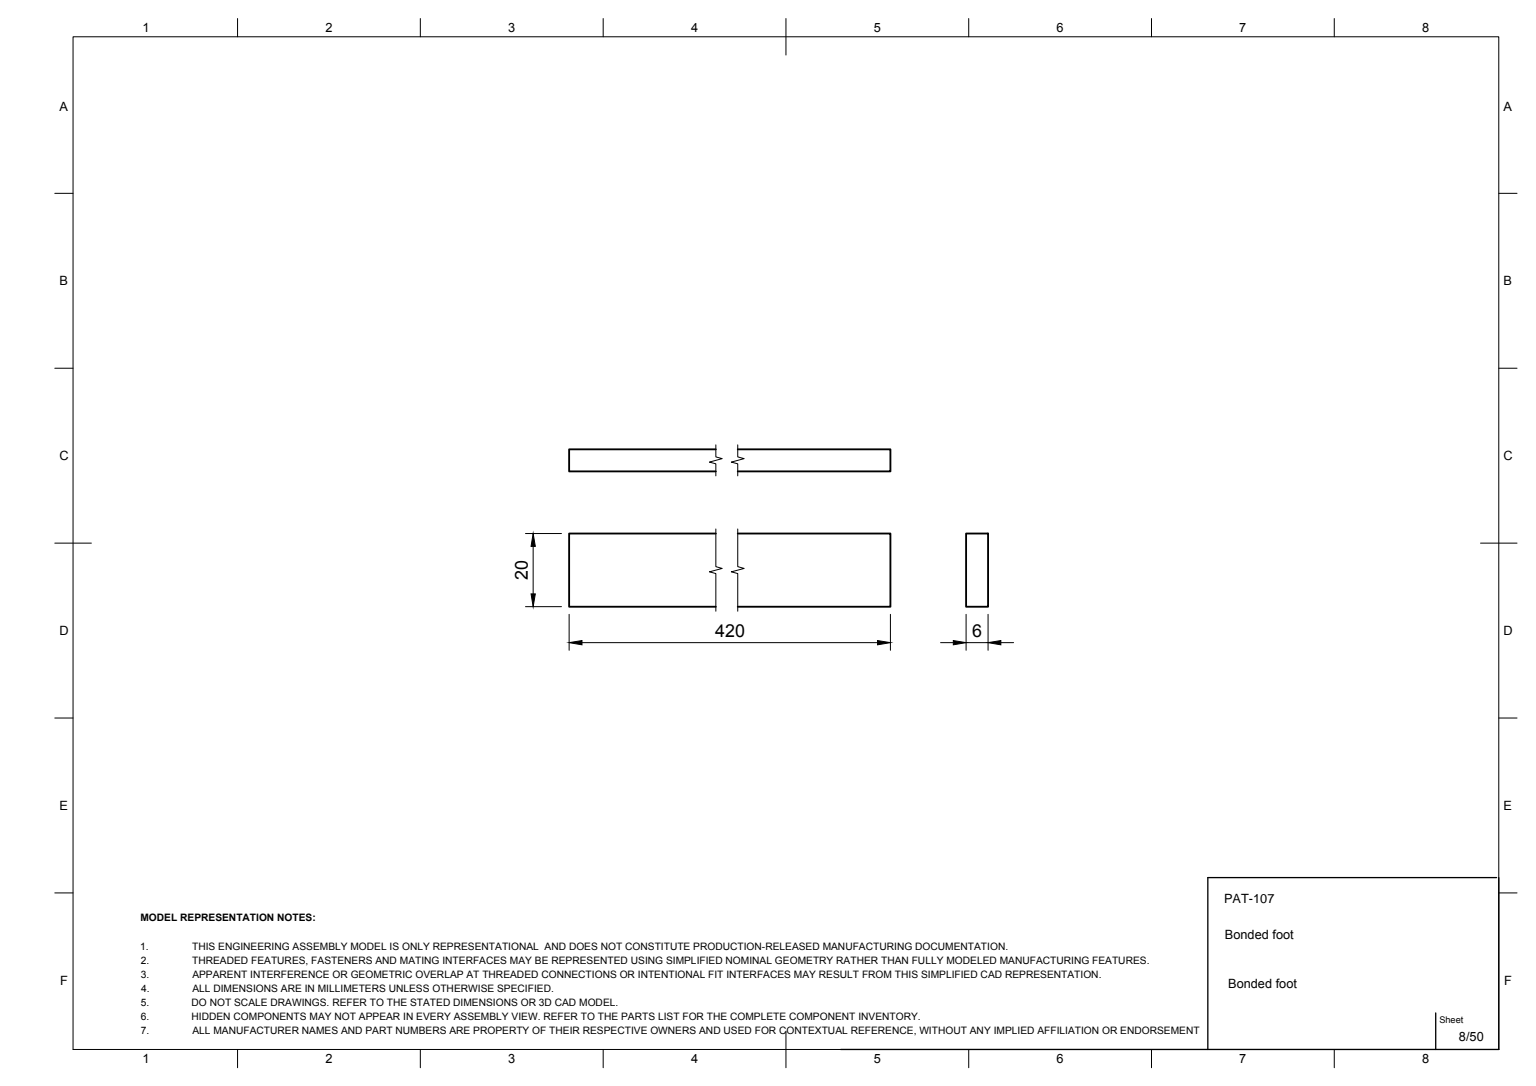
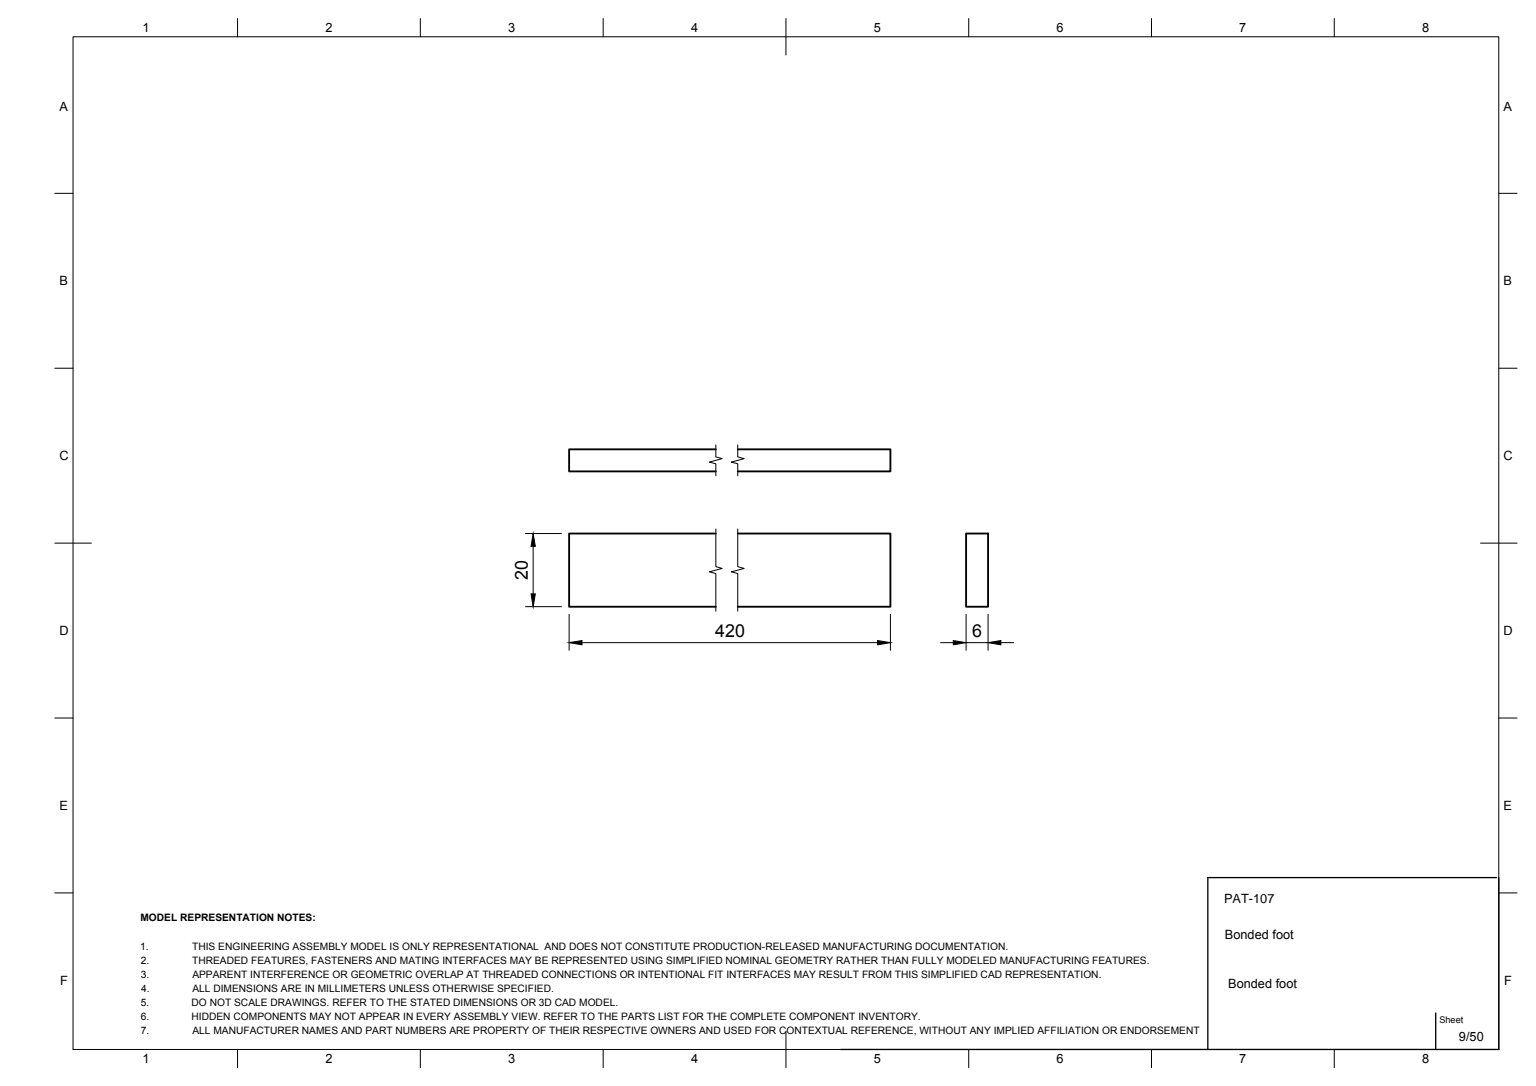
ISO-10303-21;
HEADER;
/* Generated by software containing ST-Developer
 * from STEP Tools, Inc. (www.steptools.com) 
 */

FILE_DESCRIPTION(
/* description */ ('Turntable on roller ring'),
/* implementation_level */ '2;1');

FILE_NAME(
/* name */ 'Bonded foot.step',
/* time_stamp */ '2026-10-28T03:23:59-07:00',
/* author */ (''),
/* organization */ (''),
/* preprocessor_version */ 'ST-DEVELOPER v20.2',
/* originating_system */ 'Autodesk Translation Framework v15.17.0.0',
/* authorisation */ '');

FILE_SCHEMA (('AUTOMOTIVE_DESIGN { 1 0 10303 214 3 1 1 }'));
ENDSEC;

DATA;
#10=MECHANICAL_DESIGN_GEOMETRIC_PRESENTATION_REPRESENTATION('',(#635),#16281);
#516=SHAPE_REPRESENTATION_RELATIONSHIP('SRR','None',#16531,#571);
#571=ADVANCED_BREP_SHAPE_REPRESENTATION('',(#706),#16225);
#635=STYLED_ITEM('',(#16946),#706);
#706=MANIFOLD_SOLID_BREP('Body1',#8377);
#1039=PLANE('',#9375);
#1040=PLANE('',#9376);
#1041=PLANE('',#9377);
#1042=PLANE('',#9378);
#1043=PLANE('',#9379);
#1044=PLANE('',#9380);
#1386=FACE_OUTER_BOUND('',#1967,.T.);
#1387=FACE_OUTER_BOUND('',#1968,.T.);
#1388=FACE_OUTER_BOUND('',#1969,.T.);
#1389=FACE_OUTER_BOUND('',#1970,.T.);
#1390=FACE_OUTER_BOUND('',#1971,.T.);
#1391=FACE_OUTER_BOUND('',#1972,.T.);
#1967=EDGE_LOOP('',(#6245,#6246,#6247,#6248));
#1968=EDGE_LOOP('',(#6249,#6250,#6251,#6252));
#1969=EDGE_LOOP('',(#6253,#6254,#6255,#6256));
#1970=EDGE_LOOP('',(#6257,#6258,#6259,#6260));
#1971=EDGE_LOOP('',(#6261,#6262,#6263,#6264));
#1972=EDGE_LOOP('',(#6265,#6266,#6267,#6268));
#2594=LINE('',#14042,#3077);
#2595=LINE('',#14044,#3078);
#2596=LINE('',#14046,#3079);
#2597=LINE('',#14047,#3080);
#2598=LINE('',#14050,#3081);
#2599=LINE('',#14052,#3082);
#2600=LINE('',#14053,#3083);
#2601=LINE('',#14056,#3084);
#2602=LINE('',#14058,#3085);
#2603=LINE('',#14059,#3086);
#2604=LINE('',#14061,#3087);
#2605=LINE('',#14062,#3088);
#3077=VECTOR('',#10973,1.);
#3078=VECTOR('',#10974,1.);
#3079=VECTOR('',#10975,1.);
#3080=VECTOR('',#10976,1.);
#3081=VECTOR('',#10979,1.);
#3082=VECTOR('',#10980,1.);
#3083=VECTOR('',#10981,1.);
#3084=VECTOR('',#10984,1.);
#3085=VECTOR('',#10985,1.);
#3086=VECTOR('',#10986,1.);
#3087=VECTOR('',#10989,1.);
#3088=VECTOR('',#10990,1.);
#4153=VERTEX_POINT('',#14040);
#4154=VERTEX_POINT('',#14041);
#4155=VERTEX_POINT('',#14043);
#4156=VERTEX_POINT('',#14045);
#4157=VERTEX_POINT('',#14049);
#4158=VERTEX_POINT('',#14051);
#4159=VERTEX_POINT('',#14055);
#4160=VERTEX_POINT('',#14057);
#4933=EDGE_CURVE('',#4153,#4154,#2594,.T.);
#4934=EDGE_CURVE('',#4154,#4155,#2595,.T.);
#4935=EDGE_CURVE('',#4156,#4155,#2596,.T.);
#4936=EDGE_CURVE('',#4153,#4156,#2597,.T.);
#4937=EDGE_CURVE('',#4157,#4153,#2598,.T.);
#4938=EDGE_CURVE('',#4158,#4156,#2599,.T.);
#4939=EDGE_CURVE('',#4157,#4158,#2600,.T.);
#4940=EDGE_CURVE('',#4159,#4157,#2601,.T.);
#4941=EDGE_CURVE('',#4160,#4158,#2602,.T.);
#4942=EDGE_CURVE('',#4159,#4160,#2603,.T.);
#4943=EDGE_CURVE('',#4154,#4159,#2604,.T.);
#4944=EDGE_CURVE('',#4155,#4160,#2605,.T.);
#6245=ORIENTED_EDGE('',*,*,#4933,.T.);
#6246=ORIENTED_EDGE('',*,*,#4934,.T.);
#6247=ORIENTED_EDGE('',*,*,#4935,.F.);
#6248=ORIENTED_EDGE('',*,*,#4936,.F.);
#6249=ORIENTED_EDGE('',*,*,#4937,.T.);
#6250=ORIENTED_EDGE('',*,*,#4936,.T.);
#6251=ORIENTED_EDGE('',*,*,#4938,.F.);
#6252=ORIENTED_EDGE('',*,*,#4939,.F.);
#6253=ORIENTED_EDGE('',*,*,#4940,.T.);
#6254=ORIENTED_EDGE('',*,*,#4939,.T.);
#6255=ORIENTED_EDGE('',*,*,#4941,.F.);
#6256=ORIENTED_EDGE('',*,*,#4942,.F.);
#6257=ORIENTED_EDGE('',*,*,#4943,.T.);
#6258=ORIENTED_EDGE('',*,*,#4942,.T.);
#6259=ORIENTED_EDGE('',*,*,#4944,.F.);
#6260=ORIENTED_EDGE('',*,*,#4934,.F.);
#6261=ORIENTED_EDGE('',*,*,#4944,.T.);
#6262=ORIENTED_EDGE('',*,*,#4941,.T.);
#6263=ORIENTED_EDGE('',*,*,#4938,.T.);
#6264=ORIENTED_EDGE('',*,*,#4935,.T.);
#6265=ORIENTED_EDGE('',*,*,#4943,.F.);
#6266=ORIENTED_EDGE('',*,*,#4933,.F.);
#6267=ORIENTED_EDGE('',*,*,#4937,.F.);
#6268=ORIENTED_EDGE('',*,*,#4940,.F.);
#7989=ADVANCED_FACE('',(#1386),#1039,.T.);
#7990=ADVANCED_FACE('',(#1387),#1040,.T.);
#7991=ADVANCED_FACE('',(#1388),#1041,.T.);
#7992=ADVANCED_FACE('',(#1389),#1042,.T.);
#7993=ADVANCED_FACE('',(#1390),#1043,.T.);
#7994=ADVANCED_FACE('',(#1391),#1044,.F.);
#8377=CLOSED_SHELL('',(#7989,#7990,#7991,#7992,#7993,#7994));
#9374=AXIS2_PLACEMENT_3D('',#14038,#10969,#10970);
#9375=AXIS2_PLACEMENT_3D('',#14039,#10971,#10972);
#9376=AXIS2_PLACEMENT_3D('',#14048,#10977,#10978);
#9377=AXIS2_PLACEMENT_3D('',#14054,#10982,#10983);
#9378=AXIS2_PLACEMENT_3D('',#14060,#10987,#10988);
#9379=AXIS2_PLACEMENT_3D('',#14063,#10991,#10992);
#9380=AXIS2_PLACEMENT_3D('',#14064,#10993,#10994);
#10969=DIRECTION('axis',(0.,0.,1.));
#10970=DIRECTION('refdir',(1.,0.,0.));
#10971=DIRECTION('center_axis',(0.,1.,0.));
#10972=DIRECTION('ref_axis',(-1.,0.,0.));
#10973=DIRECTION('',(-1.,0.,0.));
#10974=DIRECTION('',(0.,0.,1.));
#10975=DIRECTION('',(-1.,0.,0.));
#10976=DIRECTION('',(0.,0.,1.));
#10977=DIRECTION('center_axis',(1.,0.,0.));
#10978=DIRECTION('ref_axis',(0.,1.,0.));
#10979=DIRECTION('',(0.,1.,0.));
#10980=DIRECTION('',(0.,1.,0.));
#10981=DIRECTION('',(0.,0.,1.));
#10982=DIRECTION('center_axis',(0.,-1.,0.));
#10983=DIRECTION('ref_axis',(1.,0.,0.));
#10984=DIRECTION('',(1.,0.,0.));
#10985=DIRECTION('',(1.,0.,0.));
#10986=DIRECTION('',(0.,0.,1.));
#10987=DIRECTION('center_axis',(-1.,0.,0.));
#10988=DIRECTION('ref_axis',(0.,-1.,0.));
#10989=DIRECTION('',(0.,-1.,0.));
#10990=DIRECTION('',(0.,-1.,0.));
#10991=DIRECTION('center_axis',(0.,0.,1.));
#10992=DIRECTION('ref_axis',(1.,0.,0.));
#10993=DIRECTION('center_axis',(0.,0.,1.));
#10994=DIRECTION('ref_axis',(1.,0.,0.));
#14038=CARTESIAN_POINT('',(0.,0.,0.));
#14039=CARTESIAN_POINT('Origin',(-18.,21.,-0.6));
#14040=CARTESIAN_POINT('',(-18.,21.,-0.6));
#14041=CARTESIAN_POINT('',(-20.,21.,-0.6));
#14042=CARTESIAN_POINT('',(-18.,21.,-0.6));
#14043=CARTESIAN_POINT('',(-20.,21.,0.));
#14044=CARTESIAN_POINT('',(-20.,21.,-0.6));
#14045=CARTESIAN_POINT('',(-18.,21.,0.));
#14046=CARTESIAN_POINT('',(-18.,21.,0.));
#14047=CARTESIAN_POINT('',(-18.,21.,-0.6));
#14048=CARTESIAN_POINT('Origin',(-18.,-21.,-0.6));
#14049=CARTESIAN_POINT('',(-18.,-21.,-0.6));
#14050=CARTESIAN_POINT('',(-18.,-21.,-0.6));
#14051=CARTESIAN_POINT('',(-18.,-21.,0.));
#14052=CARTESIAN_POINT('',(-18.,-21.,0.));
#14053=CARTESIAN_POINT('',(-18.,-21.,-0.6));
#14054=CARTESIAN_POINT('Origin',(-20.,-21.,-0.6));
#14055=CARTESIAN_POINT('',(-20.,-21.,-0.6));
#14056=CARTESIAN_POINT('',(-20.,-21.,-0.6));
#14057=CARTESIAN_POINT('',(-20.,-21.,0.));
#14058=CARTESIAN_POINT('',(-20.,-21.,0.));
#14059=CARTESIAN_POINT('',(-20.,-21.,-0.6));
#14060=CARTESIAN_POINT('Origin',(-20.,21.,-0.6));
#14061=CARTESIAN_POINT('',(-20.,21.,-0.6));
#14062=CARTESIAN_POINT('',(-20.,21.,0.));
#14063=CARTESIAN_POINT('Origin',(-19.,0.,0.));
#14064=CARTESIAN_POINT('Origin',(-19.,0.,-0.6));
#16156=UNCERTAINTY_MEASURE_WITH_UNIT(LENGTH_MEASURE(0.001),#16282,
'DISTANCE_ACCURACY_VALUE',
'Maximum model space distance between geometric entities at asserted c
onnectivities');
#16212=UNCERTAINTY_MEASURE_WITH_UNIT(LENGTH_MEASURE(0.001),#16282,
'DISTANCE_ACCURACY_VALUE',
'Maximum model space distance between geometric entities at asserted c
onnectivities');
#16225=(
GEOMETRIC_REPRESENTATION_CONTEXT(3)
GLOBAL_UNCERTAINTY_ASSIGNED_CONTEXT((#16156))
GLOBAL_UNIT_ASSIGNED_CONTEXT((#16282,#16284,#16285))
REPRESENTATION_CONTEXT('','3D')
);
#16281=(
GEOMETRIC_REPRESENTATION_CONTEXT(3)
GLOBAL_UNCERTAINTY_ASSIGNED_CONTEXT((#16212))
GLOBAL_UNIT_ASSIGNED_CONTEXT((#16282,#16284,#16285))
REPRESENTATION_CONTEXT('','3D')
);
#16282=(
LENGTH_UNIT()
NAMED_UNIT(*)
SI_UNIT(.CENTI.,.METRE.)
);
#16284=(
NAMED_UNIT(*)
PLANE_ANGLE_UNIT()
SI_UNIT($,.RADIAN.)
);
#16285=(
NAMED_UNIT(*)
SI_UNIT($,.STERADIAN.)
SOLID_ANGLE_UNIT()
);
#16298=SHAPE_DEFINITION_REPRESENTATION(#16371,#16531);
#16371=PRODUCT_DEFINITION_SHAPE('',$,#16600);
#16531=SHAPE_REPRESENTATION('',(#9374),#16225);
#16587=PRODUCT_DEFINITION_CONTEXT('part definition',#16793,'design');
#16600=PRODUCT_DEFINITION('Bonded foot','Bonded foot',#16668,#16587);
#16668=PRODUCT_DEFINITION_FORMATION('',$,#16807);
#16793=APPLICATION_CONTEXT(
'Core Data for Automotive Mechanical Design Process');
#16794=PRODUCT_CONTEXT('part definition',#16793,'mechanical');
#16807=PRODUCT('Bonded foot','Bonded foot','Bonded foot',(#16794));
#16940=COLOUR_RGB('Off White',0.89,0.88,0.83);
#16941=FILL_AREA_STYLE_COLOUR('',#16940);
#16942=FILL_AREA_STYLE('',(#16941));
#16943=SURFACE_STYLE_FILL_AREA(#16942);
#16944=SURFACE_SIDE_STYLE('',(#16943));
#16945=SURFACE_STYLE_USAGE(.BOTH.,#16944);
#16946=PRESENTATION_STYLE_ASSIGNMENT((#16945));
ENDSEC;
END-ISO-10303-21;
